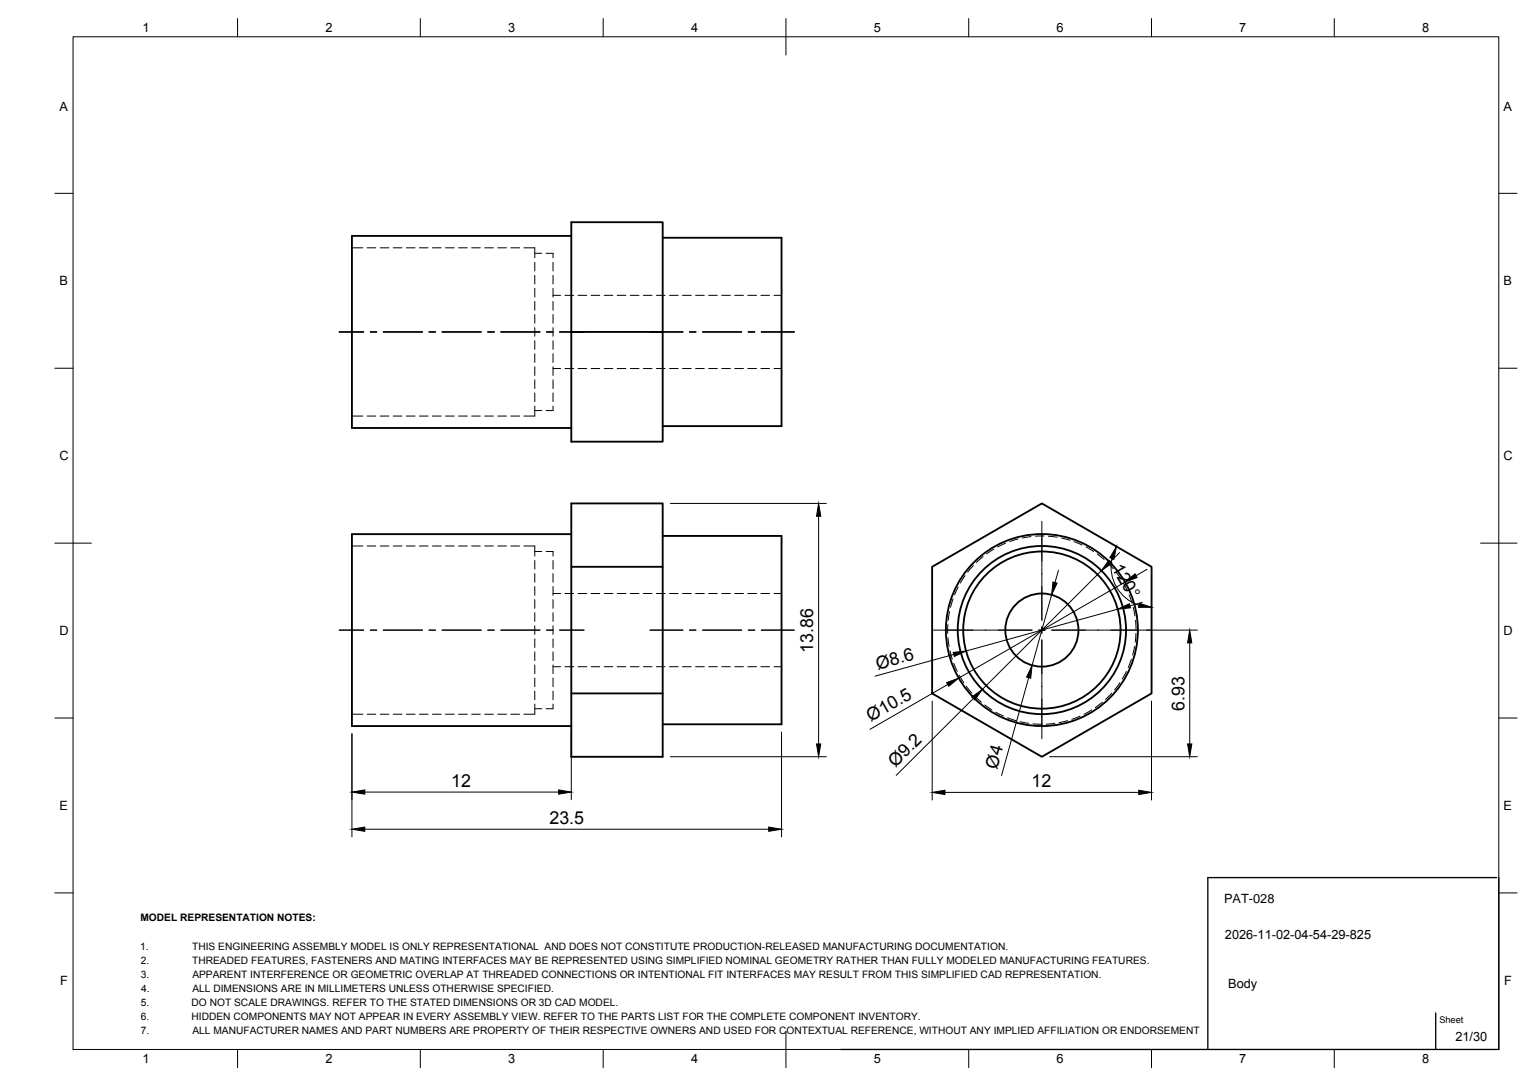
ISO-10303-21;
HEADER;
/* Generated by software containing ST-Developer
 * from STEP Tools, Inc. (www.steptools.com) 
 */

FILE_DESCRIPTION(
/* description */ ('Cylinder foot and clevis mount kit'),
/* implementation_level */ '2;1');

FILE_NAME(
/* name */ 'Body.step',
/* time_stamp */ '2026-10-27T20:10:43-07:00',
/* author */ (''),
/* organization */ (''),
/* preprocessor_version */ 'ST-DEVELOPER v20.2',
/* originating_system */ 'Autodesk Translation Framework v15.17.0.0',
/* authorisation */ '');

FILE_SCHEMA (('AUTOMOTIVE_DESIGN { 1 0 10303 214 3 1 1 }'));
ENDSEC;

DATA;
#10=MECHANICAL_DESIGN_GEOMETRIC_PRESENTATION_REPRESENTATION('',(#349),#9102);
#293=SHAPE_REPRESENTATION_RELATIONSHIP('SRR','None',#9241,#321);
#321=ADVANCED_BREP_SHAPE_REPRESENTATION('',(#376),#9084);
#349=STYLED_ITEM('',(#9439),#376);
#376=MANIFOLD_SOLID_BREP('Body1',#4936);
#457=FACE_BOUND('',#1244,.T.);
#458=FACE_BOUND('',#1246,.T.);
#459=FACE_BOUND('',#1248,.T.);
#460=FACE_BOUND('',#1256,.T.);
#461=FACE_BOUND('',#1259,.T.);
#462=FACE_BOUND('',#1263,.T.);
#616=PLANE('',#5599);
#617=PLANE('',#5601);
#618=PLANE('',#5603);
#619=PLANE('',#5605);
#620=PLANE('',#5606);
#621=PLANE('',#5607);
#622=PLANE('',#5608);
#623=PLANE('',#5609);
#624=PLANE('',#5610);
#625=PLANE('',#5611);
#626=PLANE('',#5615);
#627=PLANE('',#5620);
#871=FACE_OUTER_BOUND('',#1242,.T.);
#872=FACE_OUTER_BOUND('',#1243,.T.);
#873=FACE_OUTER_BOUND('',#1245,.T.);
#874=FACE_OUTER_BOUND('',#1247,.T.);
#875=FACE_OUTER_BOUND('',#1249,.T.);
#876=FACE_OUTER_BOUND('',#1250,.T.);
#877=FACE_OUTER_BOUND('',#1251,.T.);
#878=FACE_OUTER_BOUND('',#1252,.T.);
#879=FACE_OUTER_BOUND('',#1253,.T.);
#880=FACE_OUTER_BOUND('',#1254,.T.);
#881=FACE_OUTER_BOUND('',#1255,.T.);
#882=FACE_OUTER_BOUND('',#1257,.T.);
#883=FACE_OUTER_BOUND('',#1258,.T.);
#884=FACE_OUTER_BOUND('',#1260,.T.);
#885=FACE_OUTER_BOUND('',#1261,.T.);
#886=FACE_OUTER_BOUND('',#1262,.T.);
#887=FACE_OUTER_BOUND('',#1264,.T.);
#1242=EDGE_LOOP('',(#4021,#4022,#4023,#4024));
#1243=EDGE_LOOP('',(#4025));
#1244=EDGE_LOOP('',(#4026));
#1245=EDGE_LOOP('',(#4027,#4028,#4029,#4030,#4031,#4032));
#1246=EDGE_LOOP('',(#4033));
#1247=EDGE_LOOP('',(#4034,#4035,#4036,#4037,#4038,#4039));
#1248=EDGE_LOOP('',(#4040));
#1249=EDGE_LOOP('',(#4041,#4042,#4043,#4044));
#1250=EDGE_LOOP('',(#4045,#4046,#4047,#4048));
#1251=EDGE_LOOP('',(#4049,#4050,#4051,#4052));
#1252=EDGE_LOOP('',(#4053,#4054,#4055,#4056));
#1253=EDGE_LOOP('',(#4057,#4058,#4059,#4060));
#1254=EDGE_LOOP('',(#4061,#4062,#4063,#4064));
#1255=EDGE_LOOP('',(#4065));
#1256=EDGE_LOOP('',(#4066));
#1257=EDGE_LOOP('',(#4067,#4068,#4069,#4070));
#1258=EDGE_LOOP('',(#4071));
#1259=EDGE_LOOP('',(#4072));
#1260=EDGE_LOOP('',(#4073,#4074,#4075,#4076));
#1261=EDGE_LOOP('',(#4077,#4078,#4079,#4080));
#1262=EDGE_LOOP('',(#4081));
#1263=EDGE_LOOP('',(#4082));
#1264=EDGE_LOOP('',(#4083,#4084,#4085,#4086));
#1621=LINE('',#8266,#1970);
#1622=LINE('',#8274,#1971);
#1623=LINE('',#8276,#1972);
#1624=LINE('',#8278,#1973);
#1625=LINE('',#8280,#1974);
#1626=LINE('',#8282,#1975);
#1627=LINE('',#8283,#1976);
#1628=LINE('',#8289,#1977);
#1629=LINE('',#8291,#1978);
#1630=LINE('',#8293,#1979);
#1631=LINE('',#8295,#1980);
#1632=LINE('',#8297,#1981);
#1633=LINE('',#8298,#1982);
#1634=LINE('',#8302,#1983);
#1635=LINE('',#8303,#1984);
#1636=LINE('',#8305,#1985);
#1637=LINE('',#8307,#1986);
#1638=LINE('',#8309,#1987);
#1639=LINE('',#8311,#1988);
#1640=LINE('',#8318,#1989);
#1641=LINE('',#8324,#1990);
#1642=LINE('',#8328,#1991);
#1643=LINE('',#8333,#1992);
#1970=VECTOR('',#6772,0.43);
#1971=VECTOR('',#6781,1.);
#1972=VECTOR('',#6782,1.);
#1973=VECTOR('',#6783,1.);
#1974=VECTOR('',#6784,1.);
#1975=VECTOR('',#6785,1.);
#1976=VECTOR('',#6786,1.);
#1977=VECTOR('',#6791,1.);
#1978=VECTOR('',#6792,1.);
#1979=VECTOR('',#6793,1.);
#1980=VECTOR('',#6794,1.);
#1981=VECTOR('',#6795,1.);
#1982=VECTOR('',#6796,1.);
#1983=VECTOR('',#6801,1.);
#1984=VECTOR('',#6802,1.);
#1985=VECTOR('',#6805,1.);
#1986=VECTOR('',#6808,1.);
#1987=VECTOR('',#6811,1.);
#1988=VECTOR('',#6814,1.);
#1989=VECTOR('',#6823,0.46);
#1990=VECTOR('',#6832,0.525);
#1991=VECTOR('',#6837,0.515);
#1992=VECTOR('',#6844,0.2);
#2236=CIRCLE('',#5597,0.43);
#2237=CIRCLE('',#5598,0.43);
#2238=CIRCLE('',#5600,0.2);
#2239=CIRCLE('',#5602,0.525);
#2240=CIRCLE('',#5604,0.515);
#2241=CIRCLE('',#5612,0.46);
#2242=CIRCLE('',#5614,0.46);
#2243=CIRCLE('',#5616,0.525);
#2244=CIRCLE('',#5619,0.515);
#2245=CIRCLE('',#5621,0.2);
#2550=VERTEX_POINT('',#8263);
#2551=VERTEX_POINT('',#8265);
#2552=VERTEX_POINT('',#8269);
#2553=VERTEX_POINT('',#8272);
#2554=VERTEX_POINT('',#8273);
#2555=VERTEX_POINT('',#8275);
#2556=VERTEX_POINT('',#8277);
#2557=VERTEX_POINT('',#8279);
#2558=VERTEX_POINT('',#8281);
#2559=VERTEX_POINT('',#8284);
#2560=VERTEX_POINT('',#8287);
#2561=VERTEX_POINT('',#8288);
#2562=VERTEX_POINT('',#8290);
#2563=VERTEX_POINT('',#8292);
#2564=VERTEX_POINT('',#8294);
#2565=VERTEX_POINT('',#8296);
#2566=VERTEX_POINT('',#8299);
#2567=VERTEX_POINT('',#8314);
#2568=VERTEX_POINT('',#8317);
#2569=VERTEX_POINT('',#8321);
#2570=VERTEX_POINT('',#8326);
#2571=VERTEX_POINT('',#8330);
#3065=EDGE_CURVE('',#2550,#2550,#2236,.T.);
#3066=EDGE_CURVE('',#2550,#2551,#1621,.T.);
#3067=EDGE_CURVE('',#2551,#2551,#2237,.T.);
#3068=EDGE_CURVE('',#2552,#2552,#2238,.T.);
#3069=EDGE_CURVE('',#2553,#2554,#1622,.T.);
#3070=EDGE_CURVE('',#2554,#2555,#1623,.T.);
#3071=EDGE_CURVE('',#2555,#2556,#1624,.T.);
#3072=EDGE_CURVE('',#2556,#2557,#1625,.T.);
#3073=EDGE_CURVE('',#2557,#2558,#1626,.T.);
#3074=EDGE_CURVE('',#2558,#2553,#1627,.T.);
#3075=EDGE_CURVE('',#2559,#2559,#2239,.T.);
#3076=EDGE_CURVE('',#2560,#2561,#1628,.T.);
#3077=EDGE_CURVE('',#2562,#2560,#1629,.T.);
#3078=EDGE_CURVE('',#2563,#2562,#1630,.T.);
#3079=EDGE_CURVE('',#2564,#2563,#1631,.T.);
#3080=EDGE_CURVE('',#2565,#2564,#1632,.T.);
#3081=EDGE_CURVE('',#2561,#2565,#1633,.T.);
#3082=EDGE_CURVE('',#2566,#2566,#2240,.T.);
#3083=EDGE_CURVE('',#2560,#2553,#1634,.T.);
#3084=EDGE_CURVE('',#2562,#2558,#1635,.T.);
#3085=EDGE_CURVE('',#2563,#2557,#1636,.T.);
#3086=EDGE_CURVE('',#2564,#2556,#1637,.T.);
#3087=EDGE_CURVE('',#2565,#2555,#1638,.T.);
#3088=EDGE_CURVE('',#2561,#2554,#1639,.T.);
#3089=EDGE_CURVE('',#2567,#2567,#2241,.T.);
#3090=EDGE_CURVE('',#2567,#2568,#1640,.T.);
#3091=EDGE_CURVE('',#2568,#2568,#2242,.T.);
#3092=EDGE_CURVE('',#2569,#2569,#2243,.T.);
#3093=EDGE_CURVE('',#2559,#2569,#1641,.T.);
#3094=EDGE_CURVE('',#2570,#2570,#2244,.T.);
#3095=EDGE_CURVE('',#2570,#2566,#1642,.T.);
#3096=EDGE_CURVE('',#2571,#2571,#2245,.T.);
#3097=EDGE_CURVE('',#2571,#2552,#1643,.T.);
#4021=ORIENTED_EDGE('',*,*,#3065,.F.);
#4022=ORIENTED_EDGE('',*,*,#3066,.T.);
#4023=ORIENTED_EDGE('',*,*,#3067,.F.);
#4024=ORIENTED_EDGE('',*,*,#3066,.F.);
#4025=ORIENTED_EDGE('',*,*,#3065,.T.);
#4026=ORIENTED_EDGE('',*,*,#3068,.F.);
#4027=ORIENTED_EDGE('',*,*,#3069,.T.);
#4028=ORIENTED_EDGE('',*,*,#3070,.T.);
#4029=ORIENTED_EDGE('',*,*,#3071,.T.);
#4030=ORIENTED_EDGE('',*,*,#3072,.T.);
#4031=ORIENTED_EDGE('',*,*,#3073,.T.);
#4032=ORIENTED_EDGE('',*,*,#3074,.T.);
#4033=ORIENTED_EDGE('',*,*,#3075,.T.);
#4034=ORIENTED_EDGE('',*,*,#3076,.F.);
#4035=ORIENTED_EDGE('',*,*,#3077,.F.);
#4036=ORIENTED_EDGE('',*,*,#3078,.F.);
#4037=ORIENTED_EDGE('',*,*,#3079,.F.);
#4038=ORIENTED_EDGE('',*,*,#3080,.F.);
#4039=ORIENTED_EDGE('',*,*,#3081,.F.);
#4040=ORIENTED_EDGE('',*,*,#3082,.F.);
#4041=ORIENTED_EDGE('',*,*,#3077,.T.);
#4042=ORIENTED_EDGE('',*,*,#3083,.T.);
#4043=ORIENTED_EDGE('',*,*,#3074,.F.);
#4044=ORIENTED_EDGE('',*,*,#3084,.F.);
#4045=ORIENTED_EDGE('',*,*,#3078,.T.);
#4046=ORIENTED_EDGE('',*,*,#3084,.T.);
#4047=ORIENTED_EDGE('',*,*,#3073,.F.);
#4048=ORIENTED_EDGE('',*,*,#3085,.F.);
#4049=ORIENTED_EDGE('',*,*,#3079,.T.);
#4050=ORIENTED_EDGE('',*,*,#3085,.T.);
#4051=ORIENTED_EDGE('',*,*,#3072,.F.);
#4052=ORIENTED_EDGE('',*,*,#3086,.F.);
#4053=ORIENTED_EDGE('',*,*,#3080,.T.);
#4054=ORIENTED_EDGE('',*,*,#3086,.T.);
#4055=ORIENTED_EDGE('',*,*,#3071,.F.);
#4056=ORIENTED_EDGE('',*,*,#3087,.F.);
#4057=ORIENTED_EDGE('',*,*,#3081,.T.);
#4058=ORIENTED_EDGE('',*,*,#3087,.T.);
#4059=ORIENTED_EDGE('',*,*,#3070,.F.);
#4060=ORIENTED_EDGE('',*,*,#3088,.F.);
#4061=ORIENTED_EDGE('',*,*,#3076,.T.);
#4062=ORIENTED_EDGE('',*,*,#3088,.T.);
#4063=ORIENTED_EDGE('',*,*,#3069,.F.);
#4064=ORIENTED_EDGE('',*,*,#3083,.F.);
#4065=ORIENTED_EDGE('',*,*,#3089,.F.);
#4066=ORIENTED_EDGE('',*,*,#3067,.T.);
#4067=ORIENTED_EDGE('',*,*,#3089,.T.);
#4068=ORIENTED_EDGE('',*,*,#3090,.T.);
#4069=ORIENTED_EDGE('',*,*,#3091,.F.);
#4070=ORIENTED_EDGE('',*,*,#3090,.F.);
#4071=ORIENTED_EDGE('',*,*,#3092,.F.);
#4072=ORIENTED_EDGE('',*,*,#3091,.T.);
#4073=ORIENTED_EDGE('',*,*,#3075,.F.);
#4074=ORIENTED_EDGE('',*,*,#3093,.T.);
#4075=ORIENTED_EDGE('',*,*,#3092,.T.);
#4076=ORIENTED_EDGE('',*,*,#3093,.F.);
#4077=ORIENTED_EDGE('',*,*,#3094,.F.);
#4078=ORIENTED_EDGE('',*,*,#3095,.T.);
#4079=ORIENTED_EDGE('',*,*,#3082,.T.);
#4080=ORIENTED_EDGE('',*,*,#3095,.F.);
#4081=ORIENTED_EDGE('',*,*,#3094,.T.);
#4082=ORIENTED_EDGE('',*,*,#3096,.F.);
#4083=ORIENTED_EDGE('',*,*,#3096,.T.);
#4084=ORIENTED_EDGE('',*,*,#3097,.T.);
#4085=ORIENTED_EDGE('',*,*,#3068,.T.);
#4086=ORIENTED_EDGE('',*,*,#3097,.F.);
#4582=CYLINDRICAL_SURFACE('',#5596,0.43);
#4583=CYLINDRICAL_SURFACE('',#5613,0.46);
#4584=CYLINDRICAL_SURFACE('',#5617,0.525);
#4585=CYLINDRICAL_SURFACE('',#5618,0.515);
#4586=CYLINDRICAL_SURFACE('',#5622,0.2);
#4794=ADVANCED_FACE('',(#871),#4582,.F.);
#4795=ADVANCED_FACE('',(#872,#457),#616,.T.);
#4796=ADVANCED_FACE('',(#873,#458),#617,.T.);
#4797=ADVANCED_FACE('',(#874,#459),#618,.F.);
#4798=ADVANCED_FACE('',(#875),#619,.T.);
#4799=ADVANCED_FACE('',(#876),#620,.T.);
#4800=ADVANCED_FACE('',(#877),#621,.T.);
#4801=ADVANCED_FACE('',(#878),#622,.T.);
#4802=ADVANCED_FACE('',(#879),#623,.T.);
#4803=ADVANCED_FACE('',(#880),#624,.T.);
#4804=ADVANCED_FACE('',(#881,#460),#625,.T.);
#4805=ADVANCED_FACE('',(#882),#4583,.F.);
#4806=ADVANCED_FACE('',(#883,#461),#626,.T.);
#4807=ADVANCED_FACE('',(#884),#4584,.T.);
#4808=ADVANCED_FACE('',(#885),#4585,.T.);
#4809=ADVANCED_FACE('',(#886,#462),#627,.T.);
#4810=ADVANCED_FACE('',(#887),#4586,.F.);
#4936=CLOSED_SHELL('',(#4794,#4795,#4796,#4797,#4798,#4799,#4800,#4801,
#4802,#4803,#4804,#4805,#4806,#4807,#4808,#4809,#4810));
#5595=AXIS2_PLACEMENT_3D('',#8261,#6766,#6767);
#5596=AXIS2_PLACEMENT_3D('',#8262,#6768,#6769);
#5597=AXIS2_PLACEMENT_3D('',#8264,#6770,#6771);
#5598=AXIS2_PLACEMENT_3D('',#8267,#6773,#6774);
#5599=AXIS2_PLACEMENT_3D('',#8268,#6775,#6776);
#5600=AXIS2_PLACEMENT_3D('',#8270,#6777,#6778);
#5601=AXIS2_PLACEMENT_3D('',#8271,#6779,#6780);
#5602=AXIS2_PLACEMENT_3D('',#8285,#6787,#6788);
#5603=AXIS2_PLACEMENT_3D('',#8286,#6789,#6790);
#5604=AXIS2_PLACEMENT_3D('',#8300,#6797,#6798);
#5605=AXIS2_PLACEMENT_3D('',#8301,#6799,#6800);
#5606=AXIS2_PLACEMENT_3D('',#8304,#6803,#6804);
#5607=AXIS2_PLACEMENT_3D('',#8306,#6806,#6807);
#5608=AXIS2_PLACEMENT_3D('',#8308,#6809,#6810);
#5609=AXIS2_PLACEMENT_3D('',#8310,#6812,#6813);
#5610=AXIS2_PLACEMENT_3D('',#8312,#6815,#6816);
#5611=AXIS2_PLACEMENT_3D('',#8313,#6817,#6818);
#5612=AXIS2_PLACEMENT_3D('',#8315,#6819,#6820);
#5613=AXIS2_PLACEMENT_3D('',#8316,#6821,#6822);
#5614=AXIS2_PLACEMENT_3D('',#8319,#6824,#6825);
#5615=AXIS2_PLACEMENT_3D('',#8320,#6826,#6827);
#5616=AXIS2_PLACEMENT_3D('',#8322,#6828,#6829);
#5617=AXIS2_PLACEMENT_3D('',#8323,#6830,#6831);
#5618=AXIS2_PLACEMENT_3D('',#8325,#6833,#6834);
#5619=AXIS2_PLACEMENT_3D('',#8327,#6835,#6836);
#5620=AXIS2_PLACEMENT_3D('',#8329,#6838,#6839);
#5621=AXIS2_PLACEMENT_3D('',#8331,#6840,#6841);
#5622=AXIS2_PLACEMENT_3D('',#8332,#6842,#6843);
#6766=DIRECTION('axis',(0.,0.,1.));
#6767=DIRECTION('refdir',(1.,0.,0.));
#6768=DIRECTION('center_axis',(0.,1.,0.));
#6769=DIRECTION('ref_axis',(1.,0.,0.));
#6770=DIRECTION('center_axis',(0.,1.,0.));
#6771=DIRECTION('ref_axis',(1.,0.,0.));
#6772=DIRECTION('',(0.,1.,0.));
#6773=DIRECTION('center_axis',(0.,-1.,0.));
#6774=DIRECTION('ref_axis',(1.,0.,0.));
#6775=DIRECTION('center_axis',(0.,1.,0.));
#6776=DIRECTION('ref_axis',(1.,0.,0.));
#6777=DIRECTION('center_axis',(0.,1.,0.));
#6778=DIRECTION('ref_axis',(1.,0.,0.));
#6779=DIRECTION('center_axis',(0.,1.,0.));
#6780=DIRECTION('ref_axis',(1.,0.,0.));
#6781=DIRECTION('',(0.5,0.,-0.866025403784439));
#6782=DIRECTION('',(-0.5,0.,-0.866025403784439));
#6783=DIRECTION('',(-1.,0.,-1.60246890531964E-16));
#6784=DIRECTION('',(-0.5,0.,0.866025403784439));
#6785=DIRECTION('',(0.5,0.,0.866025403784439));
#6786=DIRECTION('',(1.,0.,1.60246890531964E-16));
#6787=DIRECTION('center_axis',(0.,-1.,0.));
#6788=DIRECTION('ref_axis',(1.,0.,0.));
#6789=DIRECTION('center_axis',(0.,1.,0.));
#6790=DIRECTION('ref_axis',(1.,0.,0.));
#6791=DIRECTION('',(0.5,0.,-0.866025403784439));
#6792=DIRECTION('',(1.,0.,1.60246890531964E-16));
#6793=DIRECTION('',(0.5,0.,0.866025403784439));
#6794=DIRECTION('',(-0.5,0.,0.866025403784439));
#6795=DIRECTION('',(-1.,0.,-1.60246890531964E-16));
#6796=DIRECTION('',(-0.5,0.,-0.866025403784439));
#6797=DIRECTION('center_axis',(0.,-1.,0.));
#6798=DIRECTION('ref_axis',(1.,0.,0.));
#6799=DIRECTION('center_axis',(-1.60246890531964E-16,0.,1.));
#6800=DIRECTION('ref_axis',(1.,0.,1.60246890531964E-16));
#6801=DIRECTION('',(0.,1.,0.));
#6802=DIRECTION('',(0.,1.,0.));
#6803=DIRECTION('center_axis',(-0.866025403784439,0.,0.5));
#6804=DIRECTION('ref_axis',(0.5,0.,0.866025403784439));
#6805=DIRECTION('',(0.,1.,0.));
#6806=DIRECTION('center_axis',(-0.866025403784439,0.,-0.5));
#6807=DIRECTION('ref_axis',(-0.5,0.,0.866025403784439));
#6808=DIRECTION('',(0.,1.,0.));
#6809=DIRECTION('center_axis',(1.60246890531964E-16,0.,-1.));
#6810=DIRECTION('ref_axis',(-1.,0.,-1.60246890531964E-16));
#6811=DIRECTION('',(0.,1.,0.));
#6812=DIRECTION('center_axis',(0.866025403784439,0.,-0.5));
#6813=DIRECTION('ref_axis',(-0.5,0.,-0.866025403784439));
#6814=DIRECTION('',(0.,1.,0.));
#6815=DIRECTION('center_axis',(0.866025403784439,0.,0.5));
#6816=DIRECTION('ref_axis',(0.5,0.,-0.866025403784439));
#6817=DIRECTION('center_axis',(0.,1.,0.));
#6818=DIRECTION('ref_axis',(0.,0.,1.));
#6819=DIRECTION('center_axis',(0.,-1.,0.));
#6820=DIRECTION('ref_axis',(1.,0.,0.));
#6821=DIRECTION('center_axis',(0.,-1.,0.));
#6822=DIRECTION('ref_axis',(1.,0.,0.));
#6823=DIRECTION('',(0.,1.,0.));
#6824=DIRECTION('center_axis',(0.,-1.,0.));
#6825=DIRECTION('ref_axis',(1.,0.,0.));
#6826=DIRECTION('center_axis',(0.,1.,0.));
#6827=DIRECTION('ref_axis',(0.,0.,1.));
#6828=DIRECTION('center_axis',(0.,-1.,0.));
#6829=DIRECTION('ref_axis',(1.,0.,0.));
#6830=DIRECTION('center_axis',(0.,-1.,0.));
#6831=DIRECTION('ref_axis',(1.,0.,0.));
#6832=DIRECTION('',(0.,1.,0.));
#6833=DIRECTION('center_axis',(0.,-1.,0.));
#6834=DIRECTION('ref_axis',(1.,0.,0.));
#6835=DIRECTION('center_axis',(0.,-1.,0.));
#6836=DIRECTION('ref_axis',(1.,0.,0.));
#6837=DIRECTION('',(0.,1.,0.));
#6838=DIRECTION('center_axis',(0.,-1.,0.));
#6839=DIRECTION('ref_axis',(0.,0.,-1.));
#6840=DIRECTION('center_axis',(0.,-1.,0.));
#6841=DIRECTION('ref_axis',(1.,0.,0.));
#6842=DIRECTION('center_axis',(0.,-1.,0.));
#6843=DIRECTION('ref_axis',(1.,0.,0.));
#6844=DIRECTION('',(0.,1.,0.));
#8261=CARTESIAN_POINT('',(0.,0.,0.));
#8262=CARTESIAN_POINT('Origin',(0.,0.6,0.));
#8263=CARTESIAN_POINT('',(-0.43,0.6,5.26598123633362E-17));
#8264=CARTESIAN_POINT('Origin',(0.,0.6,0.));
#8265=CARTESIAN_POINT('',(-0.43,0.7,-5.26598123633362E-17));
#8266=CARTESIAN_POINT('',(-0.43,0.6,5.26598123633362E-17));
#8267=CARTESIAN_POINT('Origin',(0.,0.7,0.));
#8268=CARTESIAN_POINT('Origin',(0.,0.6,0.));
#8269=CARTESIAN_POINT('',(-0.2,0.6,2.44929359829471E-17));
#8270=CARTESIAN_POINT('Origin',(0.,0.6,0.));
#8271=CARTESIAN_POINT('Origin',(0.,0.5,-1.11022302462516E-16));
#8272=CARTESIAN_POINT('',(0.346410161513776,0.5,0.6));
#8273=CARTESIAN_POINT('',(0.692820323027551,0.5,0.));
#8274=CARTESIAN_POINT('',(0.346410161513776,0.5,0.6));
#8275=CARTESIAN_POINT('',(0.346410161513776,0.5,-0.6));
#8276=CARTESIAN_POINT('',(0.692820323027551,0.5,0.));
#8277=CARTESIAN_POINT('',(-0.346410161513775,0.5,-0.6));
#8278=CARTESIAN_POINT('',(0.346410161513776,0.5,-0.6));
#8279=CARTESIAN_POINT('',(-0.692820323027551,0.5,-8.48460190979926E-17));
#8280=CARTESIAN_POINT('',(-0.346410161513775,0.5,-0.6));
#8281=CARTESIAN_POINT('',(-0.346410161513776,0.5,0.6));
#8282=CARTESIAN_POINT('',(-0.692820323027551,0.5,-8.48460190979926E-17));
#8283=CARTESIAN_POINT('',(-0.346410161513776,0.5,0.6));
#8284=CARTESIAN_POINT('',(-0.525,0.5,-6.4293956955236E-17));
#8285=CARTESIAN_POINT('Origin',(0.,0.5,0.));
#8286=CARTESIAN_POINT('Origin',(0.,0.,-1.11022302462516E-16));
#8287=CARTESIAN_POINT('',(0.346410161513776,0.,0.6));
#8288=CARTESIAN_POINT('',(0.692820323027551,0.,0.));
#8289=CARTESIAN_POINT('',(0.346410161513776,0.,0.6));
#8290=CARTESIAN_POINT('',(-0.346410161513776,0.,0.6));
#8291=CARTESIAN_POINT('',(-0.346410161513776,0.,0.6));
#8292=CARTESIAN_POINT('',(-0.692820323027551,0.,-8.48460190979926E-17));
#8293=CARTESIAN_POINT('',(-0.692820323027551,0.,-8.48460190979926E-17));
#8294=CARTESIAN_POINT('',(-0.346410161513775,0.,-0.6));
#8295=CARTESIAN_POINT('',(-0.346410161513775,0.,-0.6));
#8296=CARTESIAN_POINT('',(0.346410161513776,0.,-0.6));
#8297=CARTESIAN_POINT('',(0.346410161513776,0.,-0.6));
#8298=CARTESIAN_POINT('',(0.692820323027551,0.,0.));
#8299=CARTESIAN_POINT('',(-0.515,0.,-6.30693101560887E-17));
#8300=CARTESIAN_POINT('Origin',(0.,0.,0.));
#8301=CARTESIAN_POINT('Origin',(-0.346410161513776,0.,0.6));
#8302=CARTESIAN_POINT('',(0.346410161513776,0.,0.6));
#8303=CARTESIAN_POINT('',(-0.346410161513776,0.,0.6));
#8304=CARTESIAN_POINT('Origin',(-0.692820323027551,0.,-8.48460190979926E-17));
#8305=CARTESIAN_POINT('',(-0.692820323027551,0.,-8.48460190979926E-17));
#8306=CARTESIAN_POINT('Origin',(-0.346410161513775,0.,-0.6));
#8307=CARTESIAN_POINT('',(-0.346410161513775,0.,-0.6));
#8308=CARTESIAN_POINT('Origin',(0.346410161513776,0.,-0.6));
#8309=CARTESIAN_POINT('',(0.346410161513776,0.,-0.6));
#8310=CARTESIAN_POINT('Origin',(0.692820323027551,0.,0.));
#8311=CARTESIAN_POINT('',(0.692820323027551,0.,0.));
#8312=CARTESIAN_POINT('Origin',(0.346410161513776,0.,0.6));
#8313=CARTESIAN_POINT('Origin',(0.46,0.7,0.));
#8314=CARTESIAN_POINT('',(-0.46,0.7,-5.63337527607782E-17));
#8315=CARTESIAN_POINT('Origin',(0.,0.7,0.));
#8316=CARTESIAN_POINT('Origin',(0.,1.2,0.));
#8317=CARTESIAN_POINT('',(-0.46,1.7,-5.63337527607782E-17));
#8318=CARTESIAN_POINT('',(-0.46,1.2,-5.63337527607782E-17));
#8319=CARTESIAN_POINT('Origin',(0.,1.7,0.));
#8320=CARTESIAN_POINT('Origin',(0.525,1.7,0.));
#8321=CARTESIAN_POINT('',(-0.525,1.7,-6.4293956955236E-17));
#8322=CARTESIAN_POINT('Origin',(0.,1.7,0.));
#8323=CARTESIAN_POINT('Origin',(0.,1.1,0.));
#8324=CARTESIAN_POINT('',(-0.525,1.1,-6.4293956955236E-17));
#8325=CARTESIAN_POINT('Origin',(0.,-0.325,0.));
#8326=CARTESIAN_POINT('',(-0.515,-0.65,-6.30693101560887E-17));
#8327=CARTESIAN_POINT('Origin',(0.,-0.65,0.));
#8328=CARTESIAN_POINT('',(-0.515,-0.325,-6.30693101560887E-17));
#8329=CARTESIAN_POINT('Origin',(0.2,-0.65,0.));
#8330=CARTESIAN_POINT('',(-0.2,-0.65,-2.44929359829471E-17));
#8331=CARTESIAN_POINT('Origin',(0.,-0.65,0.));
#8332=CARTESIAN_POINT('Origin',(0.,0.0249999999999999,0.));
#8333=CARTESIAN_POINT('',(-0.2,0.0249999999999999,-2.44929359829471E-17));
#9051=UNCERTAINTY_MEASURE_WITH_UNIT(LENGTH_MEASURE(0.001),#9103,
'DISTANCE_ACCURACY_VALUE',
'Maximum model space distance between geometric entities at asserted c
onnectivities');
#9069=UNCERTAINTY_MEASURE_WITH_UNIT(LENGTH_MEASURE(0.001),#9103,
'DISTANCE_ACCURACY_VALUE',
'Maximum model space distance between geometric entities at asserted c
onnectivities');
#9084=(
GEOMETRIC_REPRESENTATION_CONTEXT(3)
GLOBAL_UNCERTAINTY_ASSIGNED_CONTEXT((#9051))
GLOBAL_UNIT_ASSIGNED_CONTEXT((#9103,#9105,#9106))
REPRESENTATION_CONTEXT('','3D')
);
#9102=(
GEOMETRIC_REPRESENTATION_CONTEXT(3)
GLOBAL_UNCERTAINTY_ASSIGNED_CONTEXT((#9069))
GLOBAL_UNIT_ASSIGNED_CONTEXT((#9103,#9105,#9106))
REPRESENTATION_CONTEXT('','3D')
);
#9103=(
LENGTH_UNIT()
NAMED_UNIT(*)
SI_UNIT(.CENTI.,.METRE.)
);
#9105=(
NAMED_UNIT(*)
PLANE_ANGLE_UNIT()
SI_UNIT($,.RADIAN.)
);
#9106=(
NAMED_UNIT(*)
SI_UNIT($,.STERADIAN.)
SOLID_ANGLE_UNIT()
);
#9121=SHAPE_DEFINITION_REPRESENTATION(#9153,#9241);
#9153=PRODUCT_DEFINITION_SHAPE('',$,#9274);
#9241=SHAPE_REPRESENTATION('',(#5595),#9084);
#9259=PRODUCT_DEFINITION_CONTEXT('part definition',#9357,'design');
#9274=PRODUCT_DEFINITION('Body','Body',#9306,#9259);
#9306=PRODUCT_DEFINITION_FORMATION('',$,#9373);
#9357=APPLICATION_CONTEXT(
'Core Data for Automotive Mechanical Design Process');
#9358=PRODUCT_CONTEXT('part definition',#9357,'mechanical');
#9373=PRODUCT('Body','Body','Body',(#9358));
#9433=COLOUR_RGB('Dark Blue',0.08,0.2,0.34);
#9434=FILL_AREA_STYLE_COLOUR('',#9433);
#9435=FILL_AREA_STYLE('',(#9434));
#9436=SURFACE_STYLE_FILL_AREA(#9435);
#9437=SURFACE_SIDE_STYLE('',(#9436));
#9438=SURFACE_STYLE_USAGE(.BOTH.,#9437);
#9439=PRESENTATION_STYLE_ASSIGNMENT((#9438));
ENDSEC;
END-ISO-10303-21;
